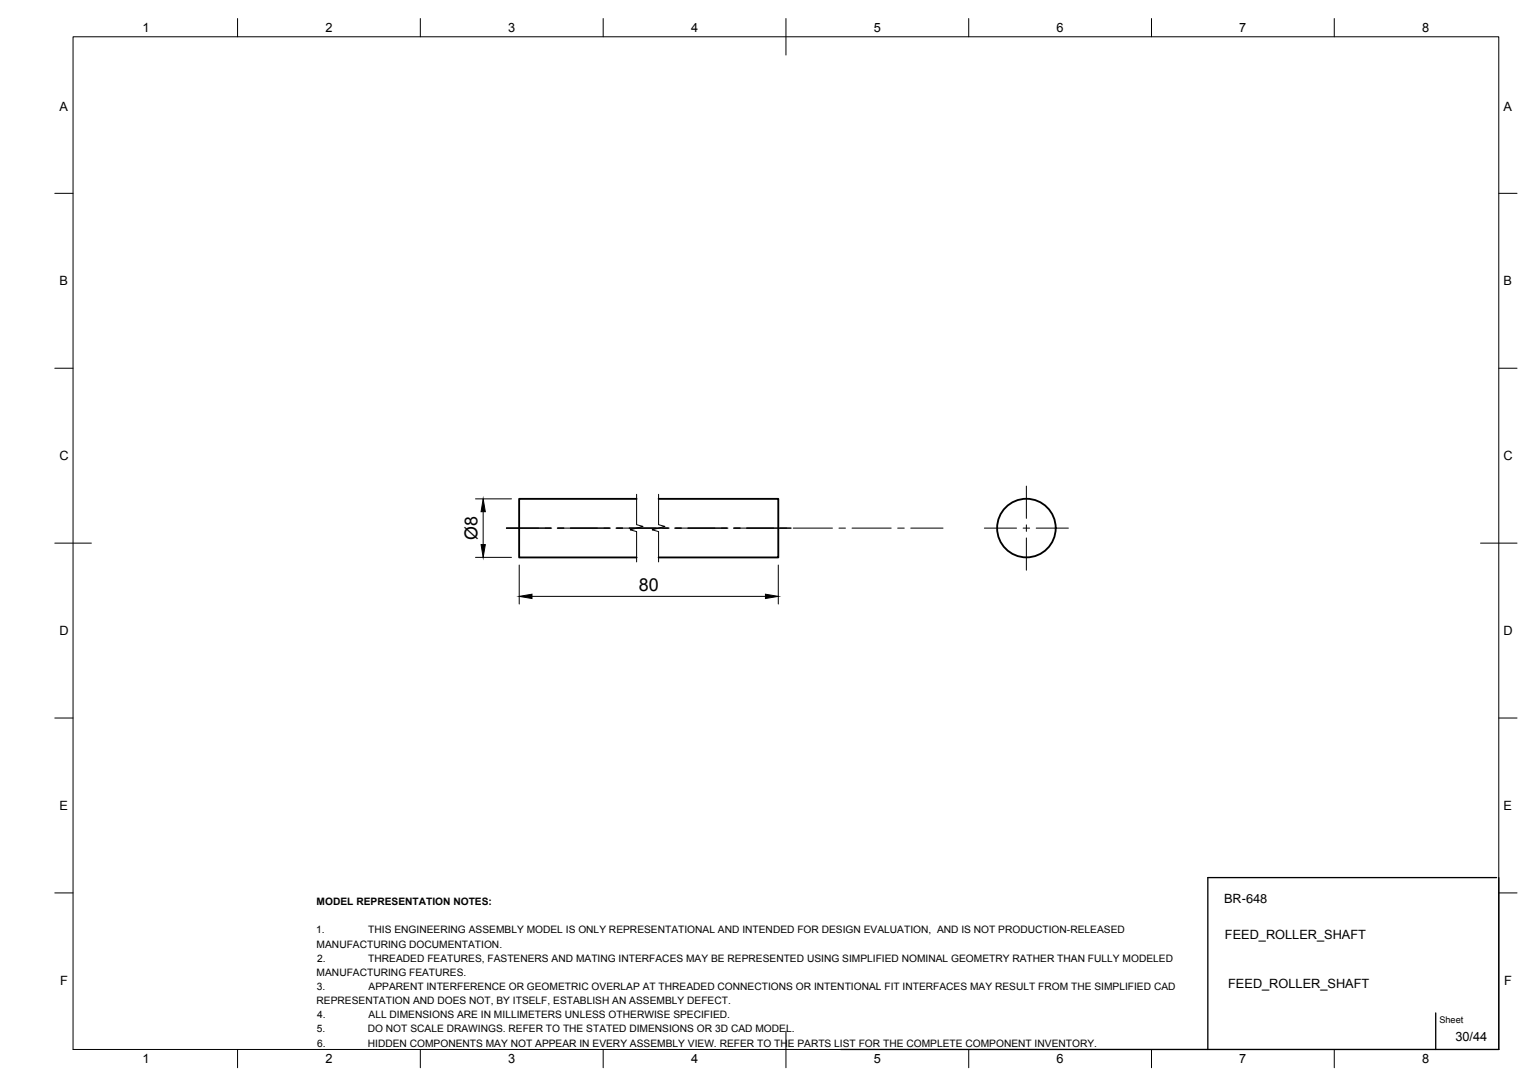
ISO-10303-21;
HEADER;
FILE_DESCRIPTION((''),'2;1');
FILE_NAME('FEED_ROLLER_SHAFT.step','2026-10-01T22:05:39-07:00',(''),(''),'','','');
FILE_SCHEMA (('AUTOMOTIVE_DESIGN { 1 0 10303 214 3 1 1 }'));
ENDSEC;
DATA;
#10=MECHANICAL_DESIGN_GEOMETRIC_PRESENTATION_REPRESENTATION('',(#628),#24628);
#544=SHAPE_REPRESENTATION_RELATIONSHIP('SRR','None',#24817,#586) ;
#586=ADVANCED_BREP_SHAPE_REPRESENTATION('',(#667),#24607) ;
#628=STYLED_ITEM('',(#25030),#667) ;
#667=MANIFOLD_SOLID_BREP('FEED_ROLLER_SHAFT',#13170) ;
#1559=LINE('',#23286,#2395) ;
#2395=VECTOR('',#18636,0.4) ;
#2897=CYLINDRICAL_SURFACE('',#14994,0.4) ;
#3523=FACE_OUTER_BOUND('',#4490,.T.) ;
#3524=FACE_OUTER_BOUND('',#4491,.T.) ;
#3525=FACE_OUTER_BOUND('',#4492,.T.) ;
#4490=EDGE_LOOP('',(#11129,#11130,#11131,#11132)) ;
#4491=EDGE_LOOP('',(#11133)) ;
#4492=EDGE_LOOP('',(#11134)) ;
#5405=CIRCLE('',#14995,0.4) ;
#5406=CIRCLE('',#14996,0.4) ;
#6447=VERTEX_POINT('',#23283) ;
#6448=VERTEX_POINT('',#23285) ;
#8054=EDGE_CURVE('',#6447,#6447,#5405,.T.) ;
#8055=EDGE_CURVE('',#6447,#6448,#1559,.T.) ;
#8056=EDGE_CURVE('',#6448,#6448,#5406,.T.) ;
#11129=ORIENTED_EDGE('',*,*,#8054,.F.) ;
#11130=ORIENTED_EDGE('',*,*,#8055,.T.) ;
#11131=ORIENTED_EDGE('',*,*,#8056,.F.) ;
#11132=ORIENTED_EDGE('',*,*,#8055,.F.) ;
#11133=ORIENTED_EDGE('',*,*,#8056,.T.) ;
#11134=ORIENTED_EDGE('',*,*,#8054,.T.) ;
#12211=PLANE('',#14997) ;
#12212=PLANE('',#14998) ;
#12918=ADVANCED_FACE('',(#3523),#2897,.T.) ;
#12919=ADVANCED_FACE('',(#3524),#12211,.T.) ;
#12920=ADVANCED_FACE('',(#3525),#12212,.T.) ;
#13170=CLOSED_SHELL('',(#12918,#12919,#12920)) ;
#14993=AXIS2_PLACEMENT_3D('',#23281,#18630,#18631) ;
#14994=AXIS2_PLACEMENT_3D('',#23282,#18632,#18633) ;
#14995=AXIS2_PLACEMENT_3D('',#23284,#18634,#18635) ;
#14996=AXIS2_PLACEMENT_3D('',#23287,#18637,#18638) ;
#14997=AXIS2_PLACEMENT_3D('',#23288,#18639,#18640) ;
#14998=AXIS2_PLACEMENT_3D('',#23289,#18641,#18642) ;
#18630=DIRECTION('axis',(0.,0.,1.)) ;
#18631=DIRECTION('refdir',(1.,0.,0.)) ;
#18632=DIRECTION('center_axis',(0.,1.,0.)) ;
#18633=DIRECTION('ref_axis',(1.,0.,0.)) ;
#18634=DIRECTION('center_axis',(0.,1.,0.)) ;
#18635=DIRECTION('ref_axis',(1.,0.,0.)) ;
#18636=DIRECTION('',(0.,-1.,0.)) ;
#18637=DIRECTION('center_axis',(0.,-1.,0.)) ;
#18638=DIRECTION('ref_axis',(1.,0.,0.)) ;
#18639=DIRECTION('center_axis',(0.,-1.,0.)) ;
#18640=DIRECTION('ref_axis',(-1.,0.,0.)) ;
#18641=DIRECTION('center_axis',(0.,1.,0.)) ;
#18642=DIRECTION('ref_axis',(1.,0.,0.)) ;
#23281=CARTESIAN_POINT('',(0.,0.,0.)) ;
#23282=CARTESIAN_POINT('Origin',(-23.,-1.,-2.2)) ;
#23283=CARTESIAN_POINT('',(-23.4,3.,-2.2)) ;
#23284=CARTESIAN_POINT('Origin',(-23.,3.,-2.2)) ;
#23285=CARTESIAN_POINT('',(-23.4,-5.,-2.2)) ;
#23286=CARTESIAN_POINT('',(-23.4,-1.,-2.2)) ;
#23287=CARTESIAN_POINT('Origin',(-23.,-5.,-2.2)) ;
#23288=CARTESIAN_POINT('Origin',(-23.,-5.,-2.2)) ;
#23289=CARTESIAN_POINT('Origin',(-23.,3.,-2.2)) ;
#24559=UNCERTAINTY_MEASURE_WITH_UNIT(LENGTH_MEASURE(0.001),#24629,
'DISTANCE_ACCURACY_VALUE',
'Maximum model space distance between geometric entities at asserted c
onnectivities') ;
#24580=UNCERTAINTY_MEASURE_WITH_UNIT(LENGTH_MEASURE(0.001),#24629,
'DISTANCE_ACCURACY_VALUE',
'Maximum model space distance between geometric entities at asserted c
onnectivities') ;
#24607=(
GEOMETRIC_REPRESENTATION_CONTEXT(3)
GLOBAL_UNCERTAINTY_ASSIGNED_CONTEXT((#24559))
GLOBAL_UNIT_ASSIGNED_CONTEXT((#24629,#24631,#24632))
REPRESENTATION_CONTEXT('','3D')
) ;
#24628=(
GEOMETRIC_REPRESENTATION_CONTEXT(3)
GLOBAL_UNCERTAINTY_ASSIGNED_CONTEXT((#24580))
GLOBAL_UNIT_ASSIGNED_CONTEXT((#24629,#24631,#24632))
REPRESENTATION_CONTEXT('','3D')
) ;
#24629=(
LENGTH_UNIT()
NAMED_UNIT(*)
SI_UNIT(.CENTI.,.METRE.)
) ;
#24631=(
NAMED_UNIT(*)
PLANE_ANGLE_UNIT()
SI_UNIT($,.RADIAN.)
) ;
#24632=(
NAMED_UNIT(*)
SI_UNIT($,.STERADIAN.)
SOLID_ANGLE_UNIT()
) ;
#24659=SHAPE_DEFINITION_REPRESENTATION(#24728,#24817) ;
#24728=PRODUCT_DEFINITION_SHAPE('',$,#24865) ;
#24817=SHAPE_REPRESENTATION('',(#14993),#24607) ;
#24838=PRODUCT_DEFINITION_CONTEXT('part definition',#24981,'design') ;
#24865=PRODUCT_DEFINITION('FEED_ROLLER_SHAFT','FEED_ROLLER_SHAFT',
#24912,#24838) ;
#24912=PRODUCT_DEFINITION_FORMATION('',$,#25009) ;
#24981=APPLICATION_CONTEXT(
'Core Data for Automotive Mechanical Design Process') ;
#24982=PRODUCT_CONTEXT('part definition',#24981,'mechanical') ;
#25009=PRODUCT('FEED_ROLLER_SHAFT','FEED_ROLLER_SHAFT',$,(#24982)) ;
#25030=PRESENTATION_STYLE_ASSIGNMENT((#25040)) ;
#25040=SURFACE_STYLE_USAGE(.BOTH.,#25050) ;
#25050=SURFACE_SIDE_STYLE('',(#25060)) ;
#25060=SURFACE_STYLE_FILL_AREA(#25070) ;
#25070=FILL_AREA_STYLE('Steel - Satin',(#25080)) ;
#25080=FILL_AREA_STYLE_COLOUR('Steel - Satin',#25090) ;
#25090=COLOUR_RGB('Steel - Satin', 0.66274510, 0.83137255, 0.94901961) ;
ENDSEC;
END-ISO-10303-21;
